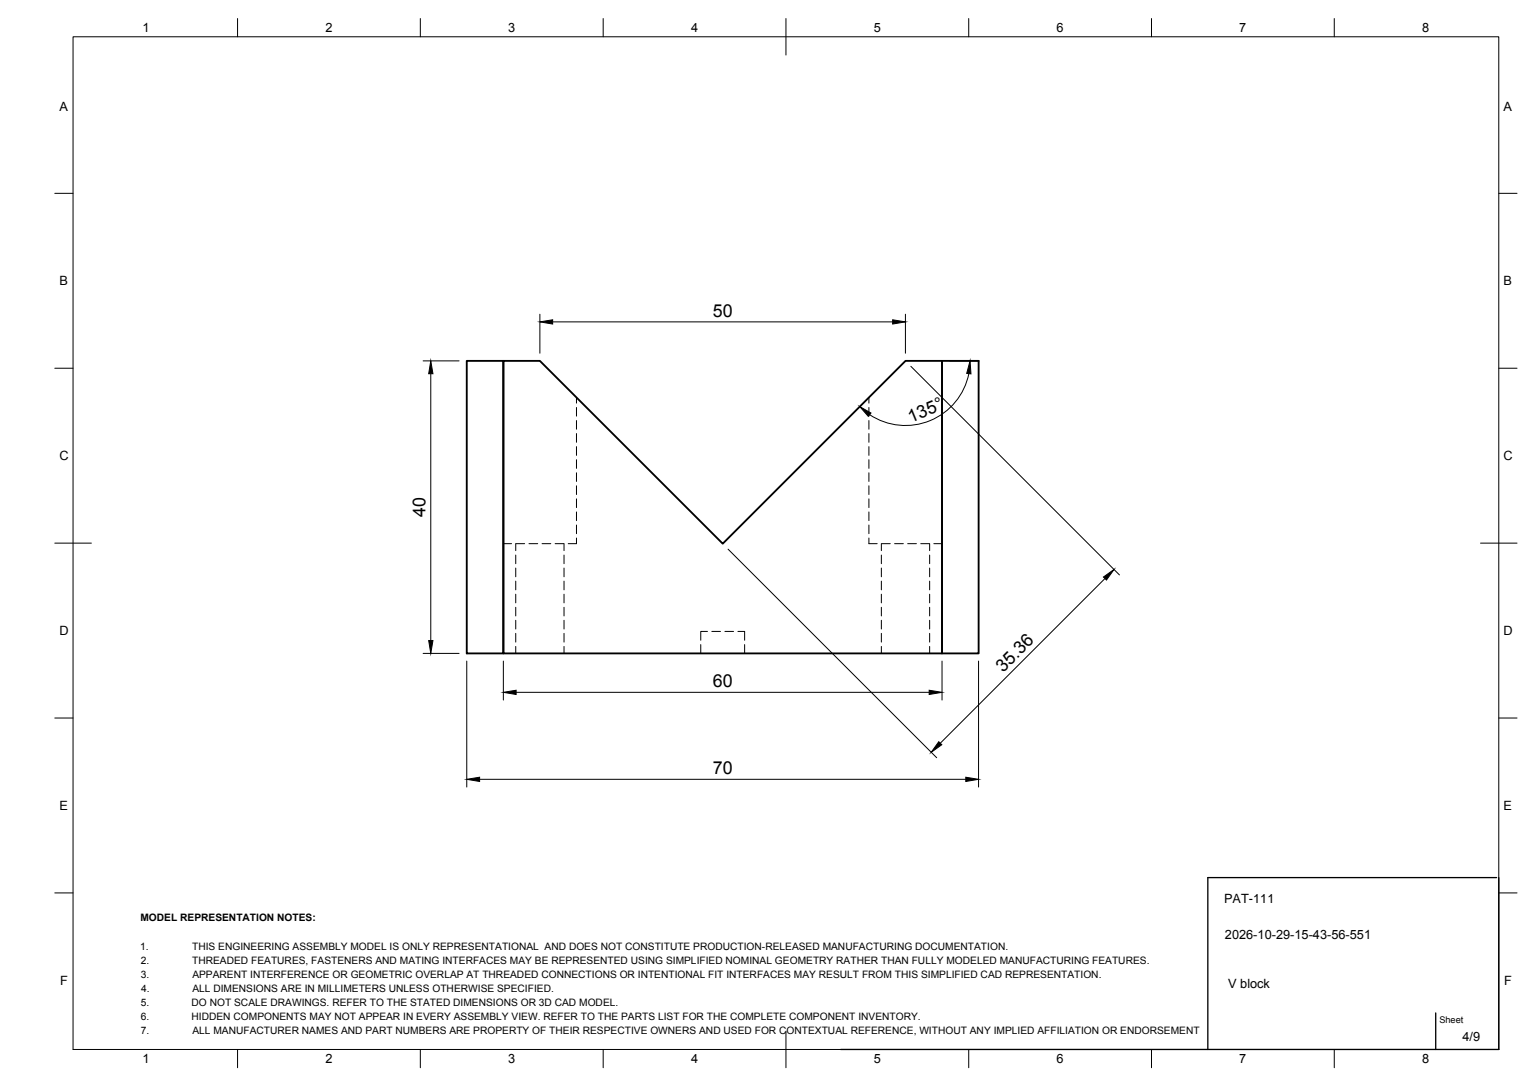
ISO-10303-21;
HEADER;
/* Generated by software containing ST-Developer
 * from STEP Tools, Inc. (www.steptools.com) 
 */

FILE_DESCRIPTION(
/* description */ ('Grid plate located blocks and clamp'),
/* implementation_level */ '2;1');

FILE_NAME(
/* name */ 'V block.step',
/* time_stamp */ '2026-10-29T15:43:47-07:00',
/* author */ (''),
/* organization */ (''),
/* preprocessor_version */ 'ST-DEVELOPER v20.2',
/* originating_system */ 'Autodesk Translation Framework v15.17.0.0',
/* authorisation */ '');

FILE_SCHEMA (('AUTOMOTIVE_DESIGN { 1 0 10303 214 3 1 1 }'));
ENDSEC;

DATA;
#10=MECHANICAL_DESIGN_GEOMETRIC_PRESENTATION_REPRESENTATION('',(#168,#169,#170),#5702);
#140=ELLIPSE('',#3521,0.707106781186547,0.5);
#141=ELLIPSE('',#3533,0.707106781186547,0.5);
#144=SHAPE_REPRESENTATION_RELATIONSHIP('SRR','None',#5762,#156);
#156=ADVANCED_BREP_SHAPE_REPRESENTATION('',(#182,#183,#184),#5692);
#168=STYLED_ITEM('',(#5876),#182);
#169=STYLED_ITEM('',(#5876),#183);
#170=STYLED_ITEM('',(#5876),#184);
#182=MANIFOLD_SOLID_BREP('Body1',#3263);
#183=MANIFOLD_SOLID_BREP('Body2',#3264);
#184=MANIFOLD_SOLID_BREP('Body3',#3265);
#244=FACE_BOUND('',#752,.T.);
#245=FACE_BOUND('',#755,.T.);
#246=FACE_BOUND('',#769,.T.);
#247=FACE_BOUND('',#770,.T.);
#248=FACE_BOUND('',#771,.T.);
#318=CIRCLE('',#3516,0.5);
#319=CIRCLE('',#3517,0.5);
#320=CIRCLE('',#3519,0.5);
#321=CIRCLE('',#3520,0.5);
#322=CIRCLE('',#3528,0.5);
#323=CIRCLE('',#3529,0.5);
#324=CIRCLE('',#3531,0.33);
#325=CIRCLE('',#3534,0.5);
#326=CIRCLE('',#3535,0.5);
#327=CIRCLE('',#3537,0.33);
#328=CIRCLE('',#3543,0.33);
#329=CIRCLE('',#3545,0.33);
#422=CYLINDRICAL_SURFACE('',#3515,0.5);
#423=CYLINDRICAL_SURFACE('',#3518,0.5);
#424=CYLINDRICAL_SURFACE('',#3527,0.5);
#425=CYLINDRICAL_SURFACE('',#3532,0.5);
#426=CYLINDRICAL_SURFACE('',#3542,0.33);
#427=CYLINDRICAL_SURFACE('',#3544,0.33);
#508=FACE_OUTER_BOUND('',#743,.T.);
#509=FACE_OUTER_BOUND('',#744,.T.);
#510=FACE_OUTER_BOUND('',#745,.T.);
#511=FACE_OUTER_BOUND('',#746,.T.);
#512=FACE_OUTER_BOUND('',#747,.T.);
#513=FACE_OUTER_BOUND('',#748,.T.);
#514=FACE_OUTER_BOUND('',#749,.T.);
#515=FACE_OUTER_BOUND('',#750,.T.);
#516=FACE_OUTER_BOUND('',#751,.T.);
#517=FACE_OUTER_BOUND('',#753,.T.);
#518=FACE_OUTER_BOUND('',#754,.T.);
#519=FACE_OUTER_BOUND('',#756,.T.);
#520=FACE_OUTER_BOUND('',#757,.T.);
#521=FACE_OUTER_BOUND('',#758,.T.);
#522=FACE_OUTER_BOUND('',#759,.T.);
#523=FACE_OUTER_BOUND('',#760,.T.);
#524=FACE_OUTER_BOUND('',#761,.T.);
#525=FACE_OUTER_BOUND('',#762,.T.);
#526=FACE_OUTER_BOUND('',#763,.T.);
#527=FACE_OUTER_BOUND('',#764,.T.);
#528=FACE_OUTER_BOUND('',#765,.T.);
#529=FACE_OUTER_BOUND('',#766,.T.);
#530=FACE_OUTER_BOUND('',#767,.T.);
#531=FACE_OUTER_BOUND('',#768,.T.);
#532=FACE_OUTER_BOUND('',#772,.T.);
#533=FACE_OUTER_BOUND('',#773,.T.);
#534=FACE_OUTER_BOUND('',#774,.T.);
#535=FACE_OUTER_BOUND('',#775,.T.);
#536=FACE_OUTER_BOUND('',#776,.T.);
#537=FACE_OUTER_BOUND('',#777,.T.);
#538=FACE_OUTER_BOUND('',#778,.T.);
#539=FACE_OUTER_BOUND('',#779,.T.);
#540=FACE_OUTER_BOUND('',#780,.T.);
#541=FACE_OUTER_BOUND('',#781,.T.);
#542=FACE_OUTER_BOUND('',#782,.T.);
#543=FACE_OUTER_BOUND('',#783,.T.);
#743=EDGE_LOOP('',(#2402,#2403,#2404,#2405));
#744=EDGE_LOOP('',(#2406,#2407,#2408,#2409,#2410));
#745=EDGE_LOOP('',(#2411,#2412,#2413,#2414));
#746=EDGE_LOOP('',(#2415,#2416,#2417,#2418));
#747=EDGE_LOOP('',(#2419,#2420,#2421,#2422));
#748=EDGE_LOOP('',(#2423,#2424,#2425,#2426));
#749=EDGE_LOOP('',(#2427,#2428,#2429,#2430));
#750=EDGE_LOOP('',(#2431,#2432,#2433,#2434));
#751=EDGE_LOOP('',(#2435,#2436));
#752=EDGE_LOOP('',(#2437));
#753=EDGE_LOOP('',(#2438,#2439,#2440,#2441,#2442));
#754=EDGE_LOOP('',(#2443,#2444));
#755=EDGE_LOOP('',(#2445));
#756=EDGE_LOOP('',(#2446,#2447,#2448,#2449,#2450,#2451));
#757=EDGE_LOOP('',(#2452,#2453,#2454,#2455));
#758=EDGE_LOOP('',(#2456,#2457,#2458,#2459,#2460,#2461));
#759=EDGE_LOOP('',(#2462,#2463,#2464,#2465));
#760=EDGE_LOOP('',(#2466,#2467,#2468,#2469));
#761=EDGE_LOOP('',(#2470,#2471,#2472,#2473));
#762=EDGE_LOOP('',(#2474,#2475,#2476,#2477));
#763=EDGE_LOOP('',(#2478,#2479,#2480,#2481));
#764=EDGE_LOOP('',(#2482,#2483,#2484,#2485,#2486,#2487,#2488));
#765=EDGE_LOOP('',(#2489,#2490,#2491,#2492,#2493,#2494,#2495));
#766=EDGE_LOOP('',(#2496,#2497,#2498,#2499,#2500,#2501,#2502));
#767=EDGE_LOOP('',(#2503,#2504,#2505,#2506,#2507,#2508,#2509));
#768=EDGE_LOOP('',(#2510,#2511,#2512,#2513));
#769=EDGE_LOOP('',(#2514,#2515,#2516,#2517));
#770=EDGE_LOOP('',(#2518));
#771=EDGE_LOOP('',(#2519));
#772=EDGE_LOOP('',(#2520,#2521,#2522,#2523));
#773=EDGE_LOOP('',(#2524,#2525,#2526,#2527));
#774=EDGE_LOOP('',(#2528,#2529,#2530,#2531));
#775=EDGE_LOOP('',(#2532,#2533,#2534,#2535));
#776=EDGE_LOOP('',(#2536,#2537,#2538,#2539));
#777=EDGE_LOOP('',(#2540,#2541,#2542,#2543));
#778=EDGE_LOOP('',(#2544,#2545,#2546,#2547));
#779=EDGE_LOOP('',(#2548,#2549,#2550,#2551));
#780=EDGE_LOOP('',(#2552,#2553,#2554,#2555));
#781=EDGE_LOOP('',(#2556,#2557,#2558,#2559));
#782=EDGE_LOOP('',(#2560,#2561,#2562,#2563));
#783=EDGE_LOOP('',(#2564,#2565,#2566,#2567));
#984=LINE('',#5025,#1257);
#985=LINE('',#5029,#1258);
#986=LINE('',#5034,#1259);
#987=LINE('',#5038,#1260);
#988=LINE('',#5045,#1261);
#989=LINE('',#5047,#1262);
#990=LINE('',#5049,#1263);
#991=LINE('',#5050,#1264);
#992=LINE('',#5053,#1265);
#993=LINE('',#5055,#1266);
#994=LINE('',#5056,#1267);
#995=LINE('',#5059,#1268);
#996=LINE('',#5061,#1269);
#997=LINE('',#5062,#1270);
#998=LINE('',#5064,#1271);
#999=LINE('',#5065,#1272);
#1000=LINE('',#5069,#1273);
#1001=LINE('',#5078,#1274);
#1002=LINE('',#5085,#1275);
#1003=LINE('',#5087,#1276);
#1004=LINE('',#5089,#1277);
#1005=LINE('',#5091,#1278);
#1006=LINE('',#5092,#1279);
#1007=LINE('',#5095,#1280);
#1008=LINE('',#5096,#1281);
#1009=LINE('',#5099,#1282);
#1010=LINE('',#5100,#1283);
#1011=LINE('',#5102,#1284);
#1012=LINE('',#5103,#1285);
#1013=LINE('',#5106,#1286);
#1014=LINE('',#5107,#1287);
#1015=LINE('',#5111,#1288);
#1016=LINE('',#5115,#1289);
#1017=LINE('',#5118,#1290);
#1018=LINE('',#5119,#1291);
#1019=LINE('',#5122,#1292);
#1020=LINE('',#5123,#1293);
#1021=LINE('',#5126,#1294);
#1022=LINE('',#5128,#1295);
#1023=LINE('',#5129,#1296);
#1024=LINE('',#5132,#1297);
#1025=LINE('',#5133,#1298);
#1026=LINE('',#5136,#1299);
#1027=LINE('',#5137,#1300);
#1028=LINE('',#5139,#1301);
#1029=LINE('',#5144,#1302);
#1030=LINE('',#5146,#1303);
#1031=LINE('',#5148,#1304);
#1032=LINE('',#5149,#1305);
#1033=LINE('',#5152,#1306);
#1034=LINE('',#5154,#1307);
#1035=LINE('',#5155,#1308);
#1036=LINE('',#5158,#1309);
#1037=LINE('',#5160,#1310);
#1038=LINE('',#5161,#1311);
#1039=LINE('',#5163,#1312);
#1040=LINE('',#5164,#1313);
#1041=LINE('',#5170,#1314);
#1042=LINE('',#5172,#1315);
#1043=LINE('',#5174,#1316);
#1044=LINE('',#5175,#1317);
#1045=LINE('',#5178,#1318);
#1046=LINE('',#5180,#1319);
#1047=LINE('',#5181,#1320);
#1048=LINE('',#5184,#1321);
#1049=LINE('',#5186,#1322);
#1050=LINE('',#5187,#1323);
#1051=LINE('',#5189,#1324);
#1052=LINE('',#5190,#1325);
#1257=VECTOR('',#4060,0.5);
#1258=VECTOR('',#4063,1.);
#1259=VECTOR('',#4068,0.5);
#1260=VECTOR('',#4071,1.);
#1261=VECTOR('',#4078,1.);
#1262=VECTOR('',#4079,1.);
#1263=VECTOR('',#4080,1.);
#1264=VECTOR('',#4081,1.);
#1265=VECTOR('',#4084,1.);
#1266=VECTOR('',#4085,1.);
#1267=VECTOR('',#4086,1.);
#1268=VECTOR('',#4089,1.);
#1269=VECTOR('',#4090,1.);
#1270=VECTOR('',#4091,1.);
#1271=VECTOR('',#4094,1.);
#1272=VECTOR('',#4095,1.);
#1273=VECTOR('',#4102,1.);
#1274=VECTOR('',#4115,1.);
#1275=VECTOR('',#4124,1.);
#1276=VECTOR('',#4125,1.);
#1277=VECTOR('',#4126,1.);
#1278=VECTOR('',#4127,1.);
#1279=VECTOR('',#4128,1.);
#1280=VECTOR('',#4131,1.);
#1281=VECTOR('',#4132,1.);
#1282=VECTOR('',#4135,1.);
#1283=VECTOR('',#4136,1.);
#1284=VECTOR('',#4137,1.);
#1285=VECTOR('',#4138,1.);
#1286=VECTOR('',#4141,1.);
#1287=VECTOR('',#4142,1.);
#1288=VECTOR('',#4147,0.33);
#1289=VECTOR('',#4152,0.33);
#1290=VECTOR('',#4155,1.);
#1291=VECTOR('',#4156,1.);
#1292=VECTOR('',#4159,1.);
#1293=VECTOR('',#4160,1.);
#1294=VECTOR('',#4163,1.);
#1295=VECTOR('',#4164,1.);
#1296=VECTOR('',#4165,1.);
#1297=VECTOR('',#4168,1.);
#1298=VECTOR('',#4169,1.);
#1299=VECTOR('',#4172,1.);
#1300=VECTOR('',#4173,1.);
#1301=VECTOR('',#4176,1.);
#1302=VECTOR('',#4181,1.);
#1303=VECTOR('',#4182,1.);
#1304=VECTOR('',#4183,1.);
#1305=VECTOR('',#4184,1.);
#1306=VECTOR('',#4187,1.);
#1307=VECTOR('',#4188,1.);
#1308=VECTOR('',#4189,1.);
#1309=VECTOR('',#4192,1.);
#1310=VECTOR('',#4193,1.);
#1311=VECTOR('',#4194,1.);
#1312=VECTOR('',#4197,1.);
#1313=VECTOR('',#4198,1.);
#1314=VECTOR('',#4205,1.);
#1315=VECTOR('',#4206,1.);
#1316=VECTOR('',#4207,1.);
#1317=VECTOR('',#4208,1.);
#1318=VECTOR('',#4211,1.);
#1319=VECTOR('',#4212,1.);
#1320=VECTOR('',#4213,1.);
#1321=VECTOR('',#4216,1.);
#1322=VECTOR('',#4217,1.);
#1323=VECTOR('',#4218,1.);
#1324=VECTOR('',#4221,1.);
#1325=VECTOR('',#4222,1.);
#1535=VERTEX_POINT('',#5023);
#1536=VERTEX_POINT('',#5024);
#1537=VERTEX_POINT('',#5026);
#1538=VERTEX_POINT('',#5028);
#1539=VERTEX_POINT('',#5032);
#1540=VERTEX_POINT('',#5033);
#1541=VERTEX_POINT('',#5035);
#1542=VERTEX_POINT('',#5037);
#1543=VERTEX_POINT('',#5039);
#1544=VERTEX_POINT('',#5043);
#1545=VERTEX_POINT('',#5044);
#1546=VERTEX_POINT('',#5046);
#1547=VERTEX_POINT('',#5048);
#1548=VERTEX_POINT('',#5052);
#1549=VERTEX_POINT('',#5054);
#1550=VERTEX_POINT('',#5058);
#1551=VERTEX_POINT('',#5060);
#1552=VERTEX_POINT('',#5072);
#1553=VERTEX_POINT('',#5075);
#1554=VERTEX_POINT('',#5081);
#1555=VERTEX_POINT('',#5084);
#1556=VERTEX_POINT('',#5086);
#1557=VERTEX_POINT('',#5088);
#1558=VERTEX_POINT('',#5090);
#1559=VERTEX_POINT('',#5094);
#1560=VERTEX_POINT('',#5098);
#1561=VERTEX_POINT('',#5101);
#1562=VERTEX_POINT('',#5105);
#1563=VERTEX_POINT('',#5109);
#1564=VERTEX_POINT('',#5113);
#1565=VERTEX_POINT('',#5117);
#1566=VERTEX_POINT('',#5121);
#1567=VERTEX_POINT('',#5125);
#1568=VERTEX_POINT('',#5127);
#1569=VERTEX_POINT('',#5131);
#1570=VERTEX_POINT('',#5135);
#1571=VERTEX_POINT('',#5142);
#1572=VERTEX_POINT('',#5143);
#1573=VERTEX_POINT('',#5145);
#1574=VERTEX_POINT('',#5147);
#1575=VERTEX_POINT('',#5151);
#1576=VERTEX_POINT('',#5153);
#1577=VERTEX_POINT('',#5157);
#1578=VERTEX_POINT('',#5159);
#1579=VERTEX_POINT('',#5168);
#1580=VERTEX_POINT('',#5169);
#1581=VERTEX_POINT('',#5171);
#1582=VERTEX_POINT('',#5173);
#1583=VERTEX_POINT('',#5177);
#1584=VERTEX_POINT('',#5179);
#1585=VERTEX_POINT('',#5183);
#1586=VERTEX_POINT('',#5185);
#1851=EDGE_CURVE('',#1535,#1536,#984,.T.);
#1852=EDGE_CURVE('',#1537,#1535,#318,.T.);
#1853=EDGE_CURVE('',#1537,#1538,#985,.T.);
#1854=EDGE_CURVE('',#1536,#1538,#319,.T.);
#1855=EDGE_CURVE('',#1539,#1540,#986,.T.);
#1856=EDGE_CURVE('',#1541,#1539,#320,.T.);
#1857=EDGE_CURVE('',#1541,#1542,#987,.T.);
#1858=EDGE_CURVE('',#1543,#1542,#321,.T.);
#1859=EDGE_CURVE('',#1540,#1543,#140,.T.);
#1860=EDGE_CURVE('',#1544,#1545,#988,.T.);
#1861=EDGE_CURVE('',#1544,#1546,#989,.T.);
#1862=EDGE_CURVE('',#1546,#1547,#990,.T.);
#1863=EDGE_CURVE('',#1545,#1547,#991,.T.);
#1864=EDGE_CURVE('',#1545,#1548,#992,.T.);
#1865=EDGE_CURVE('',#1547,#1549,#993,.T.);
#1866=EDGE_CURVE('',#1548,#1549,#994,.T.);
#1867=EDGE_CURVE('',#1548,#1550,#995,.T.);
#1868=EDGE_CURVE('',#1549,#1551,#996,.T.);
#1869=EDGE_CURVE('',#1550,#1551,#997,.T.);
#1870=EDGE_CURVE('',#1550,#1544,#998,.T.);
#1871=EDGE_CURVE('',#1551,#1546,#999,.T.);
#1872=EDGE_CURVE('',#1542,#1540,#322,.T.);
#1873=EDGE_CURVE('',#1541,#1542,#1000,.T.);
#1874=EDGE_CURVE('',#1539,#1541,#323,.T.);
#1875=EDGE_CURVE('',#1552,#1552,#324,.T.);
#1876=EDGE_CURVE('',#1553,#1536,#141,.T.);
#1877=EDGE_CURVE('',#1538,#1553,#325,.T.);
#1878=EDGE_CURVE('',#1537,#1538,#1001,.T.);
#1879=EDGE_CURVE('',#1535,#1537,#326,.T.);
#1880=EDGE_CURVE('',#1554,#1554,#327,.T.);
#1881=EDGE_CURVE('',#1555,#1543,#1002,.T.);
#1882=EDGE_CURVE('',#1556,#1555,#1003,.T.);
#1883=EDGE_CURVE('',#1557,#1556,#1004,.T.);
#1884=EDGE_CURVE('',#1558,#1557,#1005,.T.);
#1885=EDGE_CURVE('',#1540,#1558,#1006,.T.);
#1886=EDGE_CURVE('',#1542,#1559,#1007,.T.);
#1887=EDGE_CURVE('',#1559,#1555,#1008,.T.);
#1888=EDGE_CURVE('',#1560,#1536,#1009,.T.);
#1889=EDGE_CURVE('',#1557,#1560,#1010,.T.);
#1890=EDGE_CURVE('',#1561,#1556,#1011,.T.);
#1891=EDGE_CURVE('',#1553,#1561,#1012,.T.);
#1892=EDGE_CURVE('',#1538,#1562,#1013,.T.);
#1893=EDGE_CURVE('',#1562,#1560,#1014,.T.);
#1894=EDGE_CURVE('',#1563,#1563,#328,.T.);
#1895=EDGE_CURVE('',#1563,#1552,#1015,.T.);
#1896=EDGE_CURVE('',#1564,#1564,#329,.T.);
#1897=EDGE_CURVE('',#1564,#1554,#1016,.T.);
#1898=EDGE_CURVE('',#1558,#1565,#1017,.T.);
#1899=EDGE_CURVE('',#1565,#1542,#1018,.T.);
#1900=EDGE_CURVE('',#1561,#1566,#1019,.T.);
#1901=EDGE_CURVE('',#1566,#1538,#1020,.T.);
#1902=EDGE_CURVE('',#1567,#1562,#1021,.T.);
#1903=EDGE_CURVE('',#1567,#1568,#1022,.T.);
#1904=EDGE_CURVE('',#1568,#1565,#1023,.T.);
#1905=EDGE_CURVE('',#1569,#1567,#1024,.T.);
#1906=EDGE_CURVE('',#1569,#1566,#1025,.T.);
#1907=EDGE_CURVE('',#1570,#1559,#1026,.T.);
#1908=EDGE_CURVE('',#1570,#1569,#1027,.T.);
#1909=EDGE_CURVE('',#1568,#1570,#1028,.T.);
#1910=EDGE_CURVE('',#1571,#1572,#1029,.T.);
#1911=EDGE_CURVE('',#1572,#1573,#1030,.T.);
#1912=EDGE_CURVE('',#1574,#1573,#1031,.T.);
#1913=EDGE_CURVE('',#1571,#1574,#1032,.T.);
#1914=EDGE_CURVE('',#1575,#1571,#1033,.T.);
#1915=EDGE_CURVE('',#1576,#1574,#1034,.T.);
#1916=EDGE_CURVE('',#1575,#1576,#1035,.T.);
#1917=EDGE_CURVE('',#1577,#1575,#1036,.T.);
#1918=EDGE_CURVE('',#1578,#1576,#1037,.T.);
#1919=EDGE_CURVE('',#1577,#1578,#1038,.T.);
#1920=EDGE_CURVE('',#1572,#1577,#1039,.T.);
#1921=EDGE_CURVE('',#1573,#1578,#1040,.T.);
#1922=EDGE_CURVE('',#1579,#1580,#1041,.T.);
#1923=EDGE_CURVE('',#1580,#1581,#1042,.T.);
#1924=EDGE_CURVE('',#1582,#1581,#1043,.T.);
#1925=EDGE_CURVE('',#1579,#1582,#1044,.T.);
#1926=EDGE_CURVE('',#1583,#1579,#1045,.T.);
#1927=EDGE_CURVE('',#1584,#1582,#1046,.T.);
#1928=EDGE_CURVE('',#1583,#1584,#1047,.T.);
#1929=EDGE_CURVE('',#1585,#1583,#1048,.T.);
#1930=EDGE_CURVE('',#1586,#1584,#1049,.T.);
#1931=EDGE_CURVE('',#1585,#1586,#1050,.T.);
#1932=EDGE_CURVE('',#1580,#1585,#1051,.T.);
#1933=EDGE_CURVE('',#1581,#1586,#1052,.T.);
#2402=ORIENTED_EDGE('',*,*,#1851,.F.);
#2403=ORIENTED_EDGE('',*,*,#1852,.F.);
#2404=ORIENTED_EDGE('',*,*,#1853,.T.);
#2405=ORIENTED_EDGE('',*,*,#1854,.F.);
#2406=ORIENTED_EDGE('',*,*,#1855,.F.);
#2407=ORIENTED_EDGE('',*,*,#1856,.F.);
#2408=ORIENTED_EDGE('',*,*,#1857,.T.);
#2409=ORIENTED_EDGE('',*,*,#1858,.F.);
#2410=ORIENTED_EDGE('',*,*,#1859,.F.);
#2411=ORIENTED_EDGE('',*,*,#1860,.F.);
#2412=ORIENTED_EDGE('',*,*,#1861,.T.);
#2413=ORIENTED_EDGE('',*,*,#1862,.T.);
#2414=ORIENTED_EDGE('',*,*,#1863,.F.);
#2415=ORIENTED_EDGE('',*,*,#1864,.F.);
#2416=ORIENTED_EDGE('',*,*,#1863,.T.);
#2417=ORIENTED_EDGE('',*,*,#1865,.T.);
#2418=ORIENTED_EDGE('',*,*,#1866,.F.);
#2419=ORIENTED_EDGE('',*,*,#1867,.F.);
#2420=ORIENTED_EDGE('',*,*,#1866,.T.);
#2421=ORIENTED_EDGE('',*,*,#1868,.T.);
#2422=ORIENTED_EDGE('',*,*,#1869,.F.);
#2423=ORIENTED_EDGE('',*,*,#1870,.F.);
#2424=ORIENTED_EDGE('',*,*,#1869,.T.);
#2425=ORIENTED_EDGE('',*,*,#1871,.T.);
#2426=ORIENTED_EDGE('',*,*,#1861,.F.);
#2427=ORIENTED_EDGE('',*,*,#1871,.F.);
#2428=ORIENTED_EDGE('',*,*,#1868,.F.);
#2429=ORIENTED_EDGE('',*,*,#1865,.F.);
#2430=ORIENTED_EDGE('',*,*,#1862,.F.);
#2431=ORIENTED_EDGE('',*,*,#1855,.T.);
#2432=ORIENTED_EDGE('',*,*,#1872,.F.);
#2433=ORIENTED_EDGE('',*,*,#1873,.F.);
#2434=ORIENTED_EDGE('',*,*,#1874,.F.);
#2435=ORIENTED_EDGE('',*,*,#1856,.T.);
#2436=ORIENTED_EDGE('',*,*,#1874,.T.);
#2437=ORIENTED_EDGE('',*,*,#1875,.F.);
#2438=ORIENTED_EDGE('',*,*,#1851,.T.);
#2439=ORIENTED_EDGE('',*,*,#1876,.F.);
#2440=ORIENTED_EDGE('',*,*,#1877,.F.);
#2441=ORIENTED_EDGE('',*,*,#1878,.F.);
#2442=ORIENTED_EDGE('',*,*,#1879,.F.);
#2443=ORIENTED_EDGE('',*,*,#1852,.T.);
#2444=ORIENTED_EDGE('',*,*,#1879,.T.);
#2445=ORIENTED_EDGE('',*,*,#1880,.F.);
#2446=ORIENTED_EDGE('',*,*,#1859,.T.);
#2447=ORIENTED_EDGE('',*,*,#1881,.F.);
#2448=ORIENTED_EDGE('',*,*,#1882,.F.);
#2449=ORIENTED_EDGE('',*,*,#1883,.F.);
#2450=ORIENTED_EDGE('',*,*,#1884,.F.);
#2451=ORIENTED_EDGE('',*,*,#1885,.F.);
#2452=ORIENTED_EDGE('',*,*,#1858,.T.);
#2453=ORIENTED_EDGE('',*,*,#1886,.T.);
#2454=ORIENTED_EDGE('',*,*,#1887,.T.);
#2455=ORIENTED_EDGE('',*,*,#1881,.T.);
#2456=ORIENTED_EDGE('',*,*,#1876,.T.);
#2457=ORIENTED_EDGE('',*,*,#1888,.F.);
#2458=ORIENTED_EDGE('',*,*,#1889,.F.);
#2459=ORIENTED_EDGE('',*,*,#1883,.T.);
#2460=ORIENTED_EDGE('',*,*,#1890,.F.);
#2461=ORIENTED_EDGE('',*,*,#1891,.F.);
#2462=ORIENTED_EDGE('',*,*,#1854,.T.);
#2463=ORIENTED_EDGE('',*,*,#1892,.T.);
#2464=ORIENTED_EDGE('',*,*,#1893,.T.);
#2465=ORIENTED_EDGE('',*,*,#1888,.T.);
#2466=ORIENTED_EDGE('',*,*,#1894,.F.);
#2467=ORIENTED_EDGE('',*,*,#1895,.T.);
#2468=ORIENTED_EDGE('',*,*,#1875,.T.);
#2469=ORIENTED_EDGE('',*,*,#1895,.F.);
#2470=ORIENTED_EDGE('',*,*,#1896,.F.);
#2471=ORIENTED_EDGE('',*,*,#1897,.T.);
#2472=ORIENTED_EDGE('',*,*,#1880,.T.);
#2473=ORIENTED_EDGE('',*,*,#1897,.F.);
#2474=ORIENTED_EDGE('',*,*,#1872,.T.);
#2475=ORIENTED_EDGE('',*,*,#1885,.T.);
#2476=ORIENTED_EDGE('',*,*,#1898,.T.);
#2477=ORIENTED_EDGE('',*,*,#1899,.T.);
#2478=ORIENTED_EDGE('',*,*,#1877,.T.);
#2479=ORIENTED_EDGE('',*,*,#1891,.T.);
#2480=ORIENTED_EDGE('',*,*,#1900,.T.);
#2481=ORIENTED_EDGE('',*,*,#1901,.T.);
#2482=ORIENTED_EDGE('',*,*,#1884,.T.);
#2483=ORIENTED_EDGE('',*,*,#1889,.T.);
#2484=ORIENTED_EDGE('',*,*,#1893,.F.);
#2485=ORIENTED_EDGE('',*,*,#1902,.F.);
#2486=ORIENTED_EDGE('',*,*,#1903,.T.);
#2487=ORIENTED_EDGE('',*,*,#1904,.T.);
#2488=ORIENTED_EDGE('',*,*,#1898,.F.);
#2489=ORIENTED_EDGE('',*,*,#1905,.T.);
#2490=ORIENTED_EDGE('',*,*,#1902,.T.);
#2491=ORIENTED_EDGE('',*,*,#1892,.F.);
#2492=ORIENTED_EDGE('',*,*,#1853,.F.);
#2493=ORIENTED_EDGE('',*,*,#1878,.T.);
#2494=ORIENTED_EDGE('',*,*,#1901,.F.);
#2495=ORIENTED_EDGE('',*,*,#1906,.F.);
#2496=ORIENTED_EDGE('',*,*,#1882,.T.);
#2497=ORIENTED_EDGE('',*,*,#1887,.F.);
#2498=ORIENTED_EDGE('',*,*,#1907,.F.);
#2499=ORIENTED_EDGE('',*,*,#1908,.T.);
#2500=ORIENTED_EDGE('',*,*,#1906,.T.);
#2501=ORIENTED_EDGE('',*,*,#1900,.F.);
#2502=ORIENTED_EDGE('',*,*,#1890,.T.);
#2503=ORIENTED_EDGE('',*,*,#1909,.T.);
#2504=ORIENTED_EDGE('',*,*,#1907,.T.);
#2505=ORIENTED_EDGE('',*,*,#1886,.F.);
#2506=ORIENTED_EDGE('',*,*,#1857,.F.);
#2507=ORIENTED_EDGE('',*,*,#1873,.T.);
#2508=ORIENTED_EDGE('',*,*,#1899,.F.);
#2509=ORIENTED_EDGE('',*,*,#1904,.F.);
#2510=ORIENTED_EDGE('',*,*,#1903,.F.);
#2511=ORIENTED_EDGE('',*,*,#1905,.F.);
#2512=ORIENTED_EDGE('',*,*,#1908,.F.);
#2513=ORIENTED_EDGE('',*,*,#1909,.F.);
#2514=ORIENTED_EDGE('',*,*,#1867,.T.);
#2515=ORIENTED_EDGE('',*,*,#1870,.T.);
#2516=ORIENTED_EDGE('',*,*,#1860,.T.);
#2517=ORIENTED_EDGE('',*,*,#1864,.T.);
#2518=ORIENTED_EDGE('',*,*,#1894,.T.);
#2519=ORIENTED_EDGE('',*,*,#1896,.T.);
#2520=ORIENTED_EDGE('',*,*,#1910,.T.);
#2521=ORIENTED_EDGE('',*,*,#1911,.T.);
#2522=ORIENTED_EDGE('',*,*,#1912,.F.);
#2523=ORIENTED_EDGE('',*,*,#1913,.F.);
#2524=ORIENTED_EDGE('',*,*,#1914,.T.);
#2525=ORIENTED_EDGE('',*,*,#1913,.T.);
#2526=ORIENTED_EDGE('',*,*,#1915,.F.);
#2527=ORIENTED_EDGE('',*,*,#1916,.F.);
#2528=ORIENTED_EDGE('',*,*,#1917,.T.);
#2529=ORIENTED_EDGE('',*,*,#1916,.T.);
#2530=ORIENTED_EDGE('',*,*,#1918,.F.);
#2531=ORIENTED_EDGE('',*,*,#1919,.F.);
#2532=ORIENTED_EDGE('',*,*,#1920,.T.);
#2533=ORIENTED_EDGE('',*,*,#1919,.T.);
#2534=ORIENTED_EDGE('',*,*,#1921,.F.);
#2535=ORIENTED_EDGE('',*,*,#1911,.F.);
#2536=ORIENTED_EDGE('',*,*,#1921,.T.);
#2537=ORIENTED_EDGE('',*,*,#1918,.T.);
#2538=ORIENTED_EDGE('',*,*,#1915,.T.);
#2539=ORIENTED_EDGE('',*,*,#1912,.T.);
#2540=ORIENTED_EDGE('',*,*,#1920,.F.);
#2541=ORIENTED_EDGE('',*,*,#1910,.F.);
#2542=ORIENTED_EDGE('',*,*,#1914,.F.);
#2543=ORIENTED_EDGE('',*,*,#1917,.F.);
#2544=ORIENTED_EDGE('',*,*,#1922,.T.);
#2545=ORIENTED_EDGE('',*,*,#1923,.T.);
#2546=ORIENTED_EDGE('',*,*,#1924,.F.);
#2547=ORIENTED_EDGE('',*,*,#1925,.F.);
#2548=ORIENTED_EDGE('',*,*,#1926,.T.);
#2549=ORIENTED_EDGE('',*,*,#1925,.T.);
#2550=ORIENTED_EDGE('',*,*,#1927,.F.);
#2551=ORIENTED_EDGE('',*,*,#1928,.F.);
#2552=ORIENTED_EDGE('',*,*,#1929,.T.);
#2553=ORIENTED_EDGE('',*,*,#1928,.T.);
#2554=ORIENTED_EDGE('',*,*,#1930,.F.);
#2555=ORIENTED_EDGE('',*,*,#1931,.F.);
#2556=ORIENTED_EDGE('',*,*,#1932,.T.);
#2557=ORIENTED_EDGE('',*,*,#1931,.T.);
#2558=ORIENTED_EDGE('',*,*,#1933,.F.);
#2559=ORIENTED_EDGE('',*,*,#1923,.F.);
#2560=ORIENTED_EDGE('',*,*,#1933,.T.);
#2561=ORIENTED_EDGE('',*,*,#1930,.T.);
#2562=ORIENTED_EDGE('',*,*,#1927,.T.);
#2563=ORIENTED_EDGE('',*,*,#1924,.T.);
#2564=ORIENTED_EDGE('',*,*,#1932,.F.);
#2565=ORIENTED_EDGE('',*,*,#1922,.F.);
#2566=ORIENTED_EDGE('',*,*,#1926,.F.);
#2567=ORIENTED_EDGE('',*,*,#1929,.F.);
#2990=PLANE('',#3522);
#2991=PLANE('',#3523);
#2992=PLANE('',#3524);
#2993=PLANE('',#3525);
#2994=PLANE('',#3526);
#2995=PLANE('',#3530);
#2996=PLANE('',#3536);
#2997=PLANE('',#3538);
#2998=PLANE('',#3539);
#2999=PLANE('',#3540);
#3000=PLANE('',#3541);
#3001=PLANE('',#3546);
#3002=PLANE('',#3547);
#3003=PLANE('',#3548);
#3004=PLANE('',#3549);
#3005=PLANE('',#3550);
#3006=PLANE('',#3551);
#3007=PLANE('',#3552);
#3008=PLANE('',#3553);
#3009=PLANE('',#3554);
#3010=PLANE('',#3555);
#3011=PLANE('',#3556);
#3012=PLANE('',#3557);
#3013=PLANE('',#3558);
#3014=PLANE('',#3559);
#3015=PLANE('',#3560);
#3016=PLANE('',#3561);
#3017=PLANE('',#3562);
#3018=PLANE('',#3563);
#3019=PLANE('',#3564);
#3129=ADVANCED_FACE('',(#508),#422,.F.);
#3130=ADVANCED_FACE('',(#509),#423,.F.);
#3131=ADVANCED_FACE('',(#510),#2990,.F.);
#3132=ADVANCED_FACE('',(#511),#2991,.F.);
#3133=ADVANCED_FACE('',(#512),#2992,.F.);
#3134=ADVANCED_FACE('',(#513),#2993,.F.);
#3135=ADVANCED_FACE('',(#514),#2994,.F.);
#3136=ADVANCED_FACE('',(#515),#424,.F.);
#3137=ADVANCED_FACE('',(#516,#244),#2995,.T.);
#3138=ADVANCED_FACE('',(#517),#425,.F.);
#3139=ADVANCED_FACE('',(#518,#245),#2996,.T.);
#3140=ADVANCED_FACE('',(#519),#2997,.F.);
#3141=ADVANCED_FACE('',(#520),#2998,.T.);
#3142=ADVANCED_FACE('',(#521),#2999,.F.);
#3143=ADVANCED_FACE('',(#522),#3000,.T.);
#3144=ADVANCED_FACE('',(#523),#426,.F.);
#3145=ADVANCED_FACE('',(#524),#427,.F.);
#3146=ADVANCED_FACE('',(#525),#3001,.T.);
#3147=ADVANCED_FACE('',(#526),#3002,.T.);
#3148=ADVANCED_FACE('',(#527),#3003,.T.);
#3149=ADVANCED_FACE('',(#528),#3004,.T.);
#3150=ADVANCED_FACE('',(#529),#3005,.T.);
#3151=ADVANCED_FACE('',(#530),#3006,.T.);
#3152=ADVANCED_FACE('',(#531,#246,#247,#248),#3007,.F.);
#3153=ADVANCED_FACE('',(#532),#3008,.T.);
#3154=ADVANCED_FACE('',(#533),#3009,.T.);
#3155=ADVANCED_FACE('',(#534),#3010,.T.);
#3156=ADVANCED_FACE('',(#535),#3011,.T.);
#3157=ADVANCED_FACE('',(#536),#3012,.T.);
#3158=ADVANCED_FACE('',(#537),#3013,.F.);
#3159=ADVANCED_FACE('',(#538),#3014,.T.);
#3160=ADVANCED_FACE('',(#539),#3015,.T.);
#3161=ADVANCED_FACE('',(#540),#3016,.T.);
#3162=ADVANCED_FACE('',(#541),#3017,.T.);
#3163=ADVANCED_FACE('',(#542),#3018,.T.);
#3164=ADVANCED_FACE('',(#543),#3019,.F.);
#3263=CLOSED_SHELL('',(#3129,#3130,#3131,#3132,#3133,#3134,#3135,#3136,
#3137,#3138,#3139,#3140,#3141,#3142,#3143,#3144,#3145,#3146,#3147,#3148,
#3149,#3150,#3151,#3152));
#3264=CLOSED_SHELL('',(#3153,#3154,#3155,#3156,#3157,#3158));
#3265=CLOSED_SHELL('',(#3159,#3160,#3161,#3162,#3163,#3164));
#3514=AXIS2_PLACEMENT_3D('',#5021,#4056,#4057);
#3515=AXIS2_PLACEMENT_3D('',#5022,#4058,#4059);
#3516=AXIS2_PLACEMENT_3D('',#5027,#4061,#4062);
#3517=AXIS2_PLACEMENT_3D('',#5030,#4064,#4065);
#3518=AXIS2_PLACEMENT_3D('',#5031,#4066,#4067);
#3519=AXIS2_PLACEMENT_3D('',#5036,#4069,#4070);
#3520=AXIS2_PLACEMENT_3D('',#5040,#4072,#4073);
#3521=AXIS2_PLACEMENT_3D('',#5041,#4074,#4075);
#3522=AXIS2_PLACEMENT_3D('',#5042,#4076,#4077);
#3523=AXIS2_PLACEMENT_3D('',#5051,#4082,#4083);
#3524=AXIS2_PLACEMENT_3D('',#5057,#4087,#4088);
#3525=AXIS2_PLACEMENT_3D('',#5063,#4092,#4093);
#3526=AXIS2_PLACEMENT_3D('',#5066,#4096,#4097);
#3527=AXIS2_PLACEMENT_3D('',#5067,#4098,#4099);
#3528=AXIS2_PLACEMENT_3D('',#5068,#4100,#4101);
#3529=AXIS2_PLACEMENT_3D('',#5070,#4103,#4104);
#3530=AXIS2_PLACEMENT_3D('',#5071,#4105,#4106);
#3531=AXIS2_PLACEMENT_3D('',#5073,#4107,#4108);
#3532=AXIS2_PLACEMENT_3D('',#5074,#4109,#4110);
#3533=AXIS2_PLACEMENT_3D('',#5076,#4111,#4112);
#3534=AXIS2_PLACEMENT_3D('',#5077,#4113,#4114);
#3535=AXIS2_PLACEMENT_3D('',#5079,#4116,#4117);
#3536=AXIS2_PLACEMENT_3D('',#5080,#4118,#4119);
#3537=AXIS2_PLACEMENT_3D('',#5082,#4120,#4121);
#3538=AXIS2_PLACEMENT_3D('',#5083,#4122,#4123);
#3539=AXIS2_PLACEMENT_3D('',#5093,#4129,#4130);
#3540=AXIS2_PLACEMENT_3D('',#5097,#4133,#4134);
#3541=AXIS2_PLACEMENT_3D('',#5104,#4139,#4140);
#3542=AXIS2_PLACEMENT_3D('',#5108,#4143,#4144);
#3543=AXIS2_PLACEMENT_3D('',#5110,#4145,#4146);
#3544=AXIS2_PLACEMENT_3D('',#5112,#4148,#4149);
#3545=AXIS2_PLACEMENT_3D('',#5114,#4150,#4151);
#3546=AXIS2_PLACEMENT_3D('',#5116,#4153,#4154);
#3547=AXIS2_PLACEMENT_3D('',#5120,#4157,#4158);
#3548=AXIS2_PLACEMENT_3D('',#5124,#4161,#4162);
#3549=AXIS2_PLACEMENT_3D('',#5130,#4166,#4167);
#3550=AXIS2_PLACEMENT_3D('',#5134,#4170,#4171);
#3551=AXIS2_PLACEMENT_3D('',#5138,#4174,#4175);
#3552=AXIS2_PLACEMENT_3D('',#5140,#4177,#4178);
#3553=AXIS2_PLACEMENT_3D('',#5141,#4179,#4180);
#3554=AXIS2_PLACEMENT_3D('',#5150,#4185,#4186);
#3555=AXIS2_PLACEMENT_3D('',#5156,#4190,#4191);
#3556=AXIS2_PLACEMENT_3D('',#5162,#4195,#4196);
#3557=AXIS2_PLACEMENT_3D('',#5165,#4199,#4200);
#3558=AXIS2_PLACEMENT_3D('',#5166,#4201,#4202);
#3559=AXIS2_PLACEMENT_3D('',#5167,#4203,#4204);
#3560=AXIS2_PLACEMENT_3D('',#5176,#4209,#4210);
#3561=AXIS2_PLACEMENT_3D('',#5182,#4214,#4215);
#3562=AXIS2_PLACEMENT_3D('',#5188,#4219,#4220);
#3563=AXIS2_PLACEMENT_3D('',#5191,#4223,#4224);
#3564=AXIS2_PLACEMENT_3D('',#5192,#4225,#4226);
#4056=DIRECTION('axis',(0.,0.,1.));
#4057=DIRECTION('refdir',(1.,0.,0.));
#4058=DIRECTION('center_axis',(0.,0.,1.));
#4059=DIRECTION('ref_axis',(1.,0.,0.));
#4060=DIRECTION('',(0.,0.,1.));
#4061=DIRECTION('center_axis',(0.,0.,1.));
#4062=DIRECTION('ref_axis',(1.,0.,0.));
#4063=DIRECTION('',(0.,0.,1.));
#4064=DIRECTION('center_axis',(0.,0.,-1.));
#4065=DIRECTION('ref_axis',(1.,0.,0.));
#4066=DIRECTION('center_axis',(0.,0.,1.));
#4067=DIRECTION('ref_axis',(1.,0.,0.));
#4068=DIRECTION('',(0.,0.,1.));
#4069=DIRECTION('center_axis',(0.,0.,1.));
#4070=DIRECTION('ref_axis',(1.,0.,0.));
#4071=DIRECTION('',(0.,0.,1.));
#4072=DIRECTION('center_axis',(0.,0.,-1.));
#4073=DIRECTION('ref_axis',(1.,0.,0.));
#4074=DIRECTION('center_axis',(0.,-0.707106781186547,-0.707106781186548));
#4075=DIRECTION('ref_axis',(0.,0.707106781186548,-0.707106781186547));
#4076=DIRECTION('center_axis',(0.,-1.,0.));
#4077=DIRECTION('ref_axis',(1.,0.,0.));
#4078=DIRECTION('',(1.,0.,0.));
#4079=DIRECTION('',(0.,0.,1.));
#4080=DIRECTION('',(1.,0.,0.));
#4081=DIRECTION('',(0.,0.,1.));
#4082=DIRECTION('center_axis',(1.,0.,0.));
#4083=DIRECTION('ref_axis',(0.,1.,0.));
#4084=DIRECTION('',(0.,1.,0.));
#4085=DIRECTION('',(0.,1.,0.));
#4086=DIRECTION('',(0.,0.,1.));
#4087=DIRECTION('center_axis',(0.,1.,0.));
#4088=DIRECTION('ref_axis',(-1.,0.,0.));
#4089=DIRECTION('',(-1.,0.,0.));
#4090=DIRECTION('',(-1.,0.,0.));
#4091=DIRECTION('',(0.,0.,1.));
#4092=DIRECTION('center_axis',(-1.,0.,0.));
#4093=DIRECTION('ref_axis',(0.,-1.,0.));
#4094=DIRECTION('',(0.,-1.,0.));
#4095=DIRECTION('',(0.,-1.,0.));
#4096=DIRECTION('center_axis',(0.,0.,1.));
#4097=DIRECTION('ref_axis',(1.,0.,0.));
#4098=DIRECTION('center_axis',(0.,0.,1.));
#4099=DIRECTION('ref_axis',(1.,0.,0.));
#4100=DIRECTION('center_axis',(0.,0.,-1.));
#4101=DIRECTION('ref_axis',(1.,0.,0.));
#4102=DIRECTION('',(0.,0.,1.));
#4103=DIRECTION('center_axis',(0.,0.,1.));
#4104=DIRECTION('ref_axis',(1.,0.,0.));
#4105=DIRECTION('center_axis',(0.,0.,1.));
#4106=DIRECTION('ref_axis',(1.,0.,0.));
#4107=DIRECTION('center_axis',(0.,0.,1.));
#4108=DIRECTION('ref_axis',(1.,0.,0.));
#4109=DIRECTION('center_axis',(0.,0.,1.));
#4110=DIRECTION('ref_axis',(1.,0.,0.));
#4111=DIRECTION('center_axis',(0.,0.707106781186547,-0.707106781186548));
#4112=DIRECTION('ref_axis',(0.,0.707106781186548,0.707106781186547));
#4113=DIRECTION('center_axis',(0.,0.,-1.));
#4114=DIRECTION('ref_axis',(1.,0.,0.));
#4115=DIRECTION('',(0.,0.,1.));
#4116=DIRECTION('center_axis',(0.,0.,1.));
#4117=DIRECTION('ref_axis',(1.,0.,0.));
#4118=DIRECTION('center_axis',(0.,0.,1.));
#4119=DIRECTION('ref_axis',(1.,0.,0.));
#4120=DIRECTION('center_axis',(0.,0.,1.));
#4121=DIRECTION('ref_axis',(1.,0.,0.));
#4122=DIRECTION('center_axis',(0.,-0.707106781186547,-0.707106781186548));
#4123=DIRECTION('ref_axis',(0.,0.707106781186548,-0.707106781186547));
#4124=DIRECTION('',(-1.,0.,0.));
#4125=DIRECTION('',(0.,-0.707106781186548,0.707106781186547));
#4126=DIRECTION('',(1.,0.,0.));
#4127=DIRECTION('',(0.,0.707106781186548,-0.707106781186547));
#4128=DIRECTION('',(-1.,0.,0.));
#4129=DIRECTION('center_axis',(0.,0.,1.));
#4130=DIRECTION('ref_axis',(1.,0.,0.));
#4131=DIRECTION('',(1.,0.,0.));
#4132=DIRECTION('',(0.,1.,0.));
#4133=DIRECTION('center_axis',(0.,0.707106781186547,-0.707106781186548));
#4134=DIRECTION('ref_axis',(0.,0.707106781186548,0.707106781186547));
#4135=DIRECTION('',(1.,0.,0.));
#4136=DIRECTION('',(0.,0.707106781186548,0.707106781186547));
#4137=DIRECTION('',(0.,-0.707106781186548,-0.707106781186547));
#4138=DIRECTION('',(1.,0.,0.));
#4139=DIRECTION('center_axis',(0.,0.,1.));
#4140=DIRECTION('ref_axis',(1.,0.,0.));
#4141=DIRECTION('',(-1.,0.,0.));
#4142=DIRECTION('',(0.,-1.,0.));
#4143=DIRECTION('center_axis',(0.,0.,1.));
#4144=DIRECTION('ref_axis',(1.,0.,0.));
#4145=DIRECTION('center_axis',(0.,0.,1.));
#4146=DIRECTION('ref_axis',(1.,0.,0.));
#4147=DIRECTION('',(0.,0.,1.));
#4148=DIRECTION('center_axis',(0.,0.,1.));
#4149=DIRECTION('ref_axis',(1.,0.,0.));
#4150=DIRECTION('center_axis',(0.,0.,1.));
#4151=DIRECTION('ref_axis',(1.,0.,0.));
#4152=DIRECTION('',(0.,0.,1.));
#4153=DIRECTION('center_axis',(0.,0.,1.));
#4154=DIRECTION('ref_axis',(1.,0.,0.));
#4155=DIRECTION('',(0.,-1.,0.));
#4156=DIRECTION('',(1.,0.,0.));
#4157=DIRECTION('center_axis',(0.,0.,1.));
#4158=DIRECTION('ref_axis',(1.,0.,0.));
#4159=DIRECTION('',(0.,1.,0.));
#4160=DIRECTION('',(-1.,0.,0.));
#4161=DIRECTION('center_axis',(-1.,0.,0.));
#4162=DIRECTION('ref_axis',(0.,-1.,0.));
#4163=DIRECTION('',(0.,0.,1.));
#4164=DIRECTION('',(0.,-1.,0.));
#4165=DIRECTION('',(0.,0.,1.));
#4166=DIRECTION('center_axis',(0.,1.,0.));
#4167=DIRECTION('ref_axis',(-1.,0.,0.));
#4168=DIRECTION('',(-1.,0.,0.));
#4169=DIRECTION('',(0.,0.,1.));
#4170=DIRECTION('center_axis',(1.,0.,0.));
#4171=DIRECTION('ref_axis',(0.,1.,0.));
#4172=DIRECTION('',(0.,0.,1.));
#4173=DIRECTION('',(0.,1.,0.));
#4174=DIRECTION('center_axis',(0.,-1.,0.));
#4175=DIRECTION('ref_axis',(1.,0.,0.));
#4176=DIRECTION('',(1.,0.,0.));
#4177=DIRECTION('center_axis',(0.,0.,1.));
#4178=DIRECTION('ref_axis',(1.,0.,0.));
#4179=DIRECTION('center_axis',(0.,0.,1.));
#4180=DIRECTION('ref_axis',(-1.,0.,0.));
#4181=DIRECTION('',(-1.,0.,0.));
#4182=DIRECTION('',(0.,-1.,0.));
#4183=DIRECTION('',(-1.,0.,0.));
#4184=DIRECTION('',(0.,-1.,0.));
#4185=DIRECTION('center_axis',(1.,0.,0.));
#4186=DIRECTION('ref_axis',(0.,0.,1.));
#4187=DIRECTION('',(0.,0.,1.));
#4188=DIRECTION('',(0.,0.,1.));
#4189=DIRECTION('',(0.,-1.,0.));
#4190=DIRECTION('center_axis',(0.,0.,-1.));
#4191=DIRECTION('ref_axis',(1.,0.,0.));
#4192=DIRECTION('',(1.,0.,0.));
#4193=DIRECTION('',(1.,0.,0.));
#4194=DIRECTION('',(0.,-1.,0.));
#4195=DIRECTION('center_axis',(-1.,0.,0.));
#4196=DIRECTION('ref_axis',(0.,0.,-1.));
#4197=DIRECTION('',(0.,0.,-1.));
#4198=DIRECTION('',(0.,0.,-1.));
#4199=DIRECTION('center_axis',(0.,-1.,0.));
#4200=DIRECTION('ref_axis',(0.,0.,-1.));
#4201=DIRECTION('center_axis',(0.,-1.,0.));
#4202=DIRECTION('ref_axis',(1.,0.,0.));
#4203=DIRECTION('center_axis',(0.,0.,1.));
#4204=DIRECTION('ref_axis',(1.,0.,0.));
#4205=DIRECTION('',(1.,0.,0.));
#4206=DIRECTION('',(0.,1.,0.));
#4207=DIRECTION('',(1.,0.,0.));
#4208=DIRECTION('',(0.,1.,0.));
#4209=DIRECTION('center_axis',(-1.,0.,0.));
#4210=DIRECTION('ref_axis',(0.,0.,1.));
#4211=DIRECTION('',(0.,0.,1.));
#4212=DIRECTION('',(0.,0.,1.));
#4213=DIRECTION('',(0.,1.,0.));
#4214=DIRECTION('center_axis',(0.,0.,-1.));
#4215=DIRECTION('ref_axis',(-1.,0.,0.));
#4216=DIRECTION('',(-1.,0.,0.));
#4217=DIRECTION('',(-1.,0.,0.));
#4218=DIRECTION('',(0.,1.,0.));
#4219=DIRECTION('center_axis',(1.,0.,0.));
#4220=DIRECTION('ref_axis',(0.,0.,-1.));
#4221=DIRECTION('',(0.,0.,-1.));
#4222=DIRECTION('',(0.,0.,-1.));
#4223=DIRECTION('center_axis',(0.,1.,0.));
#4224=DIRECTION('ref_axis',(0.,0.,1.));
#4225=DIRECTION('center_axis',(0.,1.,0.));
#4226=DIRECTION('ref_axis',(-1.,0.,0.));
#5021=CARTESIAN_POINT('',(0.,0.,0.));
#5022=CARTESIAN_POINT('Origin',(6.5,2.5,2.5));
#5023=CARTESIAN_POINT('',(6.,2.5,2.5));
#5024=CARTESIAN_POINT('',(6.,2.5,5.));
#5025=CARTESIAN_POINT('',(6.,2.5,2.5));
#5026=CARTESIAN_POINT('',(6.5,3.,2.5));
#5027=CARTESIAN_POINT('Origin',(6.5,2.5,2.5));
#5028=CARTESIAN_POINT('',(6.5,3.,5.));
#5029=CARTESIAN_POINT('',(6.5,3.,2.5));
#5030=CARTESIAN_POINT('Origin',(6.5,2.5,5.));
#5031=CARTESIAN_POINT('Origin',(6.5,-2.5,2.5));
#5032=CARTESIAN_POINT('',(6.,-2.5,2.5));
#5033=CARTESIAN_POINT('',(6.,-2.5,5.));
#5034=CARTESIAN_POINT('',(6.,-2.5,2.5));
#5035=CARTESIAN_POINT('',(6.5,-3.,2.5));
#5036=CARTESIAN_POINT('Origin',(6.5,-2.5,2.5));
#5037=CARTESIAN_POINT('',(6.5,-3.,5.));
#5038=CARTESIAN_POINT('',(6.5,-3.,2.5));
#5039=CARTESIAN_POINT('',(7.,-2.5,5.));
#5040=CARTESIAN_POINT('Origin',(6.5,-2.5,5.));
#5041=CARTESIAN_POINT('Origin',(6.5,-2.5,5.));
#5042=CARTESIAN_POINT('Origin',(5.5,-0.3,0.9));
#5043=CARTESIAN_POINT('',(5.5,-0.3,1.));
#5044=CARTESIAN_POINT('',(7.5,-0.3,1.));
#5045=CARTESIAN_POINT('',(6.,-0.3,1.));
#5046=CARTESIAN_POINT('',(5.5,-0.3,1.3));
#5047=CARTESIAN_POINT('',(5.5,-0.3,0.9));
#5048=CARTESIAN_POINT('',(7.5,-0.3,1.3));
#5049=CARTESIAN_POINT('',(5.5,-0.3,1.3));
#5050=CARTESIAN_POINT('',(7.5,-0.3,0.9));
#5051=CARTESIAN_POINT('Origin',(7.5,-0.3,0.9));
#5052=CARTESIAN_POINT('',(7.5,0.3,1.));
#5053=CARTESIAN_POINT('',(7.5,-0.15,1.));
#5054=CARTESIAN_POINT('',(7.5,0.3,1.3));
#5055=CARTESIAN_POINT('',(7.5,-0.3,1.3));
#5056=CARTESIAN_POINT('',(7.5,0.3,0.9));
#5057=CARTESIAN_POINT('Origin',(7.5,0.3,0.9));
#5058=CARTESIAN_POINT('',(5.5,0.3,1.));
#5059=CARTESIAN_POINT('',(7.,0.3,1.));
#5060=CARTESIAN_POINT('',(5.5,0.3,1.3));
#5061=CARTESIAN_POINT('',(7.5,0.3,1.3));
#5062=CARTESIAN_POINT('',(5.5,0.3,0.9));
#5063=CARTESIAN_POINT('Origin',(5.5,0.3,0.9));
#5064=CARTESIAN_POINT('',(5.5,0.15,1.));
#5065=CARTESIAN_POINT('',(5.5,0.3,1.3));
#5066=CARTESIAN_POINT('Origin',(6.5,0.,1.3));
#5067=CARTESIAN_POINT('Origin',(6.5,-2.5,2.5));
#5068=CARTESIAN_POINT('Origin',(6.5,-2.5,5.));
#5069=CARTESIAN_POINT('',(6.5,-3.,2.5));
#5070=CARTESIAN_POINT('Origin',(6.5,-2.5,2.5));
#5071=CARTESIAN_POINT('Origin',(6.5,-2.5,2.5));
#5072=CARTESIAN_POINT('',(6.17,-2.5,2.5));
#5073=CARTESIAN_POINT('Origin',(6.5,-2.5,2.5));
#5074=CARTESIAN_POINT('Origin',(6.5,2.5,2.5));
#5075=CARTESIAN_POINT('',(7.,2.5,5.));
#5076=CARTESIAN_POINT('Origin',(6.5,2.5,5.));
#5077=CARTESIAN_POINT('Origin',(6.5,2.5,5.));
#5078=CARTESIAN_POINT('',(6.5,3.,2.5));
#5079=CARTESIAN_POINT('Origin',(6.5,2.5,2.5));
#5080=CARTESIAN_POINT('Origin',(6.5,2.5,2.5));
#5081=CARTESIAN_POINT('',(6.17,2.5,2.5));
#5082=CARTESIAN_POINT('Origin',(6.5,2.5,2.5));
#5083=CARTESIAN_POINT('Origin',(4.9,-2.6,5.1));
#5084=CARTESIAN_POINT('',(8.,-2.5,5.));
#5085=CARTESIAN_POINT('',(5.7,-2.5,5.));
#5086=CARTESIAN_POINT('',(8.,0.,2.5));
#5087=CARTESIAN_POINT('',(8.,-1.675,4.175));
#5088=CARTESIAN_POINT('',(5.,0.,2.5));
#5089=CARTESIAN_POINT('',(4.9,0.,2.5));
#5090=CARTESIAN_POINT('',(5.,-2.5,5.));
#5091=CARTESIAN_POINT('',(5.,-0.175,2.675));
#5092=CARTESIAN_POINT('',(5.7,-2.5,5.));
#5093=CARTESIAN_POINT('Origin',(6.5,0.,5.));
#5094=CARTESIAN_POINT('',(8.,-3.,5.));
#5095=CARTESIAN_POINT('',(5.,-3.,5.));
#5096=CARTESIAN_POINT('',(8.,-3.,5.));
#5097=CARTESIAN_POINT('Origin',(4.9,0.,2.5));
#5098=CARTESIAN_POINT('',(5.,2.5,5.));
#5099=CARTESIAN_POINT('',(5.7,2.5,5.));
#5100=CARTESIAN_POINT('',(5.,0.375,2.875));
#5101=CARTESIAN_POINT('',(8.,2.5,5.));
#5102=CARTESIAN_POINT('',(8.,-1.125,1.375));
#5103=CARTESIAN_POINT('',(5.7,2.5,5.));
#5104=CARTESIAN_POINT('Origin',(6.5,0.,5.));
#5105=CARTESIAN_POINT('',(5.,3.,5.));
#5106=CARTESIAN_POINT('',(8.,3.,5.));
#5107=CARTESIAN_POINT('',(5.,3.,5.));
#5108=CARTESIAN_POINT('Origin',(6.5,-2.5,0.9));
#5109=CARTESIAN_POINT('',(6.17,-2.5,1.));
#5110=CARTESIAN_POINT('Origin',(6.5,-2.5,1.));
#5111=CARTESIAN_POINT('',(6.17,-2.5,0.9));
#5112=CARTESIAN_POINT('Origin',(6.5,2.5,0.9));
#5113=CARTESIAN_POINT('',(6.17,2.5,1.));
#5114=CARTESIAN_POINT('Origin',(6.5,2.5,1.));
#5115=CARTESIAN_POINT('',(6.17,2.5,0.9));
#5116=CARTESIAN_POINT('Origin',(6.5,0.,5.));
#5117=CARTESIAN_POINT('',(5.,-3.,5.));
#5118=CARTESIAN_POINT('',(5.,3.,5.));
#5119=CARTESIAN_POINT('',(5.,-3.,5.));
#5120=CARTESIAN_POINT('Origin',(6.5,0.,5.));
#5121=CARTESIAN_POINT('',(8.,3.,5.));
#5122=CARTESIAN_POINT('',(8.,-3.,5.));
#5123=CARTESIAN_POINT('',(8.,3.,5.));
#5124=CARTESIAN_POINT('Origin',(5.,3.,1.));
#5125=CARTESIAN_POINT('',(5.,3.,1.));
#5126=CARTESIAN_POINT('',(5.,3.,1.));
#5127=CARTESIAN_POINT('',(5.,-3.,1.));
#5128=CARTESIAN_POINT('',(5.,3.,1.));
#5129=CARTESIAN_POINT('',(5.,-3.,1.));
#5130=CARTESIAN_POINT('Origin',(8.,3.,1.));
#5131=CARTESIAN_POINT('',(8.,3.,1.));
#5132=CARTESIAN_POINT('',(8.,3.,1.));
#5133=CARTESIAN_POINT('',(8.,3.,1.));
#5134=CARTESIAN_POINT('Origin',(8.,-3.,1.));
#5135=CARTESIAN_POINT('',(8.,-3.,1.));
#5136=CARTESIAN_POINT('',(8.,-3.,1.));
#5137=CARTESIAN_POINT('',(8.,-3.,1.));
#5138=CARTESIAN_POINT('Origin',(5.,-3.,1.));
#5139=CARTESIAN_POINT('',(5.,-3.,1.));
#5140=CARTESIAN_POINT('Origin',(6.5,0.,1.));
#5141=CARTESIAN_POINT('Origin',(8.,-3.,5.));
#5142=CARTESIAN_POINT('',(8.,-3.,5.));
#5143=CARTESIAN_POINT('',(5.,-3.,5.));
#5144=CARTESIAN_POINT('',(8.,-3.,5.));
#5145=CARTESIAN_POINT('',(5.,-3.5,5.));
#5146=CARTESIAN_POINT('',(5.,-3.,5.));
#5147=CARTESIAN_POINT('',(8.,-3.5,5.));
#5148=CARTESIAN_POINT('',(8.,-3.5,5.));
#5149=CARTESIAN_POINT('',(8.,-3.,5.));
#5150=CARTESIAN_POINT('Origin',(8.,-3.,1.));
#5151=CARTESIAN_POINT('',(8.,-3.,1.));
#5152=CARTESIAN_POINT('',(8.,-3.,1.));
#5153=CARTESIAN_POINT('',(8.,-3.5,1.));
#5154=CARTESIAN_POINT('',(8.,-3.5,1.));
#5155=CARTESIAN_POINT('',(8.,-3.,1.));
#5156=CARTESIAN_POINT('Origin',(5.,-3.,1.));
#5157=CARTESIAN_POINT('',(5.,-3.,1.));
#5158=CARTESIAN_POINT('',(5.,-3.,1.));
#5159=CARTESIAN_POINT('',(5.,-3.5,1.));
#5160=CARTESIAN_POINT('',(5.,-3.5,1.));
#5161=CARTESIAN_POINT('',(5.,-3.,1.));
#5162=CARTESIAN_POINT('Origin',(5.,-3.,5.));
#5163=CARTESIAN_POINT('',(5.,-3.,5.));
#5164=CARTESIAN_POINT('',(5.,-3.5,5.));
#5165=CARTESIAN_POINT('Origin',(6.5,-3.5,3.));
#5166=CARTESIAN_POINT('Origin',(6.5,-3.,3.));
#5167=CARTESIAN_POINT('Origin',(5.,3.,5.));
#5168=CARTESIAN_POINT('',(5.,3.,5.));
#5169=CARTESIAN_POINT('',(8.,3.,5.));
#5170=CARTESIAN_POINT('',(5.,3.,5.));
#5171=CARTESIAN_POINT('',(8.,3.5,5.));
#5172=CARTESIAN_POINT('',(8.,3.,5.));
#5173=CARTESIAN_POINT('',(5.,3.5,5.));
#5174=CARTESIAN_POINT('',(5.,3.5,5.));
#5175=CARTESIAN_POINT('',(5.,3.,5.));
#5176=CARTESIAN_POINT('Origin',(5.,3.,1.));
#5177=CARTESIAN_POINT('',(5.,3.,1.));
#5178=CARTESIAN_POINT('',(5.,3.,1.));
#5179=CARTESIAN_POINT('',(5.,3.5,1.));
#5180=CARTESIAN_POINT('',(5.,3.5,1.));
#5181=CARTESIAN_POINT('',(5.,3.,1.));
#5182=CARTESIAN_POINT('Origin',(8.,3.,1.));
#5183=CARTESIAN_POINT('',(8.,3.,1.));
#5184=CARTESIAN_POINT('',(8.,3.,1.));
#5185=CARTESIAN_POINT('',(8.,3.5,1.));
#5186=CARTESIAN_POINT('',(8.,3.5,1.));
#5187=CARTESIAN_POINT('',(8.,3.,1.));
#5188=CARTESIAN_POINT('Origin',(8.,3.,5.));
#5189=CARTESIAN_POINT('',(8.,3.,5.));
#5190=CARTESIAN_POINT('',(8.,3.5,5.));
#5191=CARTESIAN_POINT('Origin',(6.5,3.5,3.));
#5192=CARTESIAN_POINT('Origin',(6.5,3.,3.));
#5678=UNCERTAINTY_MEASURE_WITH_UNIT(LENGTH_MEASURE(0.001),#5703,
'DISTANCE_ACCURACY_VALUE',
'Maximum model space distance between geometric entities at asserted c
onnectivities');
#5688=UNCERTAINTY_MEASURE_WITH_UNIT(LENGTH_MEASURE(0.001),#5703,
'DISTANCE_ACCURACY_VALUE',
'Maximum model space distance between geometric entities at asserted c
onnectivities');
#5692=(
GEOMETRIC_REPRESENTATION_CONTEXT(3)
GLOBAL_UNCERTAINTY_ASSIGNED_CONTEXT((#5678))
GLOBAL_UNIT_ASSIGNED_CONTEXT((#5703,#5705,#5706))
REPRESENTATION_CONTEXT('','3D')
);
#5702=(
GEOMETRIC_REPRESENTATION_CONTEXT(3)
GLOBAL_UNCERTAINTY_ASSIGNED_CONTEXT((#5688))
GLOBAL_UNIT_ASSIGNED_CONTEXT((#5703,#5705,#5706))
REPRESENTATION_CONTEXT('','3D')
);
#5703=(
LENGTH_UNIT()
NAMED_UNIT(*)
SI_UNIT(.CENTI.,.METRE.)
);
#5705=(
NAMED_UNIT(*)
PLANE_ANGLE_UNIT()
SI_UNIT($,.RADIAN.)
);
#5706=(
NAMED_UNIT(*)
SI_UNIT($,.STERADIAN.)
SOLID_ANGLE_UNIT()
);
#5710=SHAPE_DEFINITION_REPRESENTATION(#5723,#5762);
#5723=PRODUCT_DEFINITION_SHAPE('',$,#5776);
#5762=SHAPE_REPRESENTATION('',(#3514),#5692);
#5772=PRODUCT_DEFINITION_CONTEXT('part definition',#5813,'design');
#5776=PRODUCT_DEFINITION('V block','V block',#5789,#5772);
#5789=PRODUCT_DEFINITION_FORMATION('',$,#5818);
#5813=APPLICATION_CONTEXT(
'Core Data for Automotive Mechanical Design Process');
#5814=PRODUCT_CONTEXT('part definition',#5813,'mechanical');
#5818=PRODUCT('V block','V block','V block',(#5814));
#5870=COLOUR_RGB('Dark Blue',0.08,0.2,0.34);
#5871=FILL_AREA_STYLE_COLOUR('',#5870);
#5872=FILL_AREA_STYLE('',(#5871));
#5873=SURFACE_STYLE_FILL_AREA(#5872);
#5874=SURFACE_SIDE_STYLE('',(#5873));
#5875=SURFACE_STYLE_USAGE(.BOTH.,#5874);
#5876=PRESENTATION_STYLE_ASSIGNMENT((#5875));
ENDSEC;
END-ISO-10303-21;
